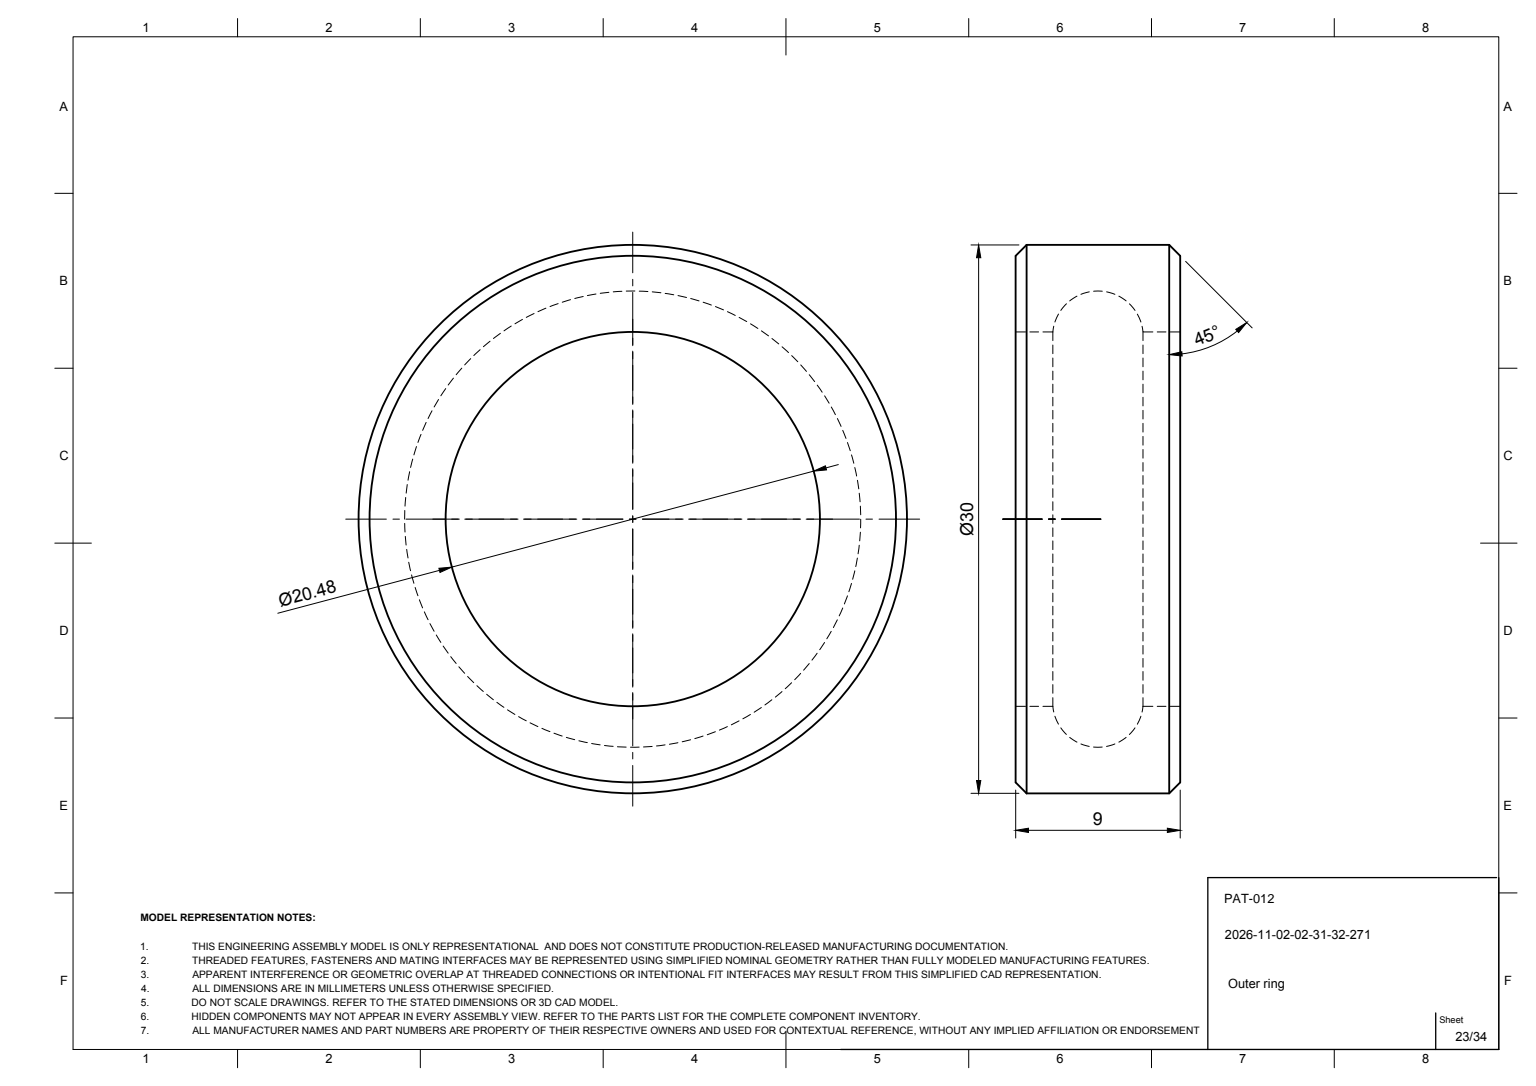
ISO-10303-21;
HEADER;
/* Generated by software containing ST-Developer
 * from STEP Tools, Inc. (www.steptools.com) 
 */

FILE_DESCRIPTION(
/* description */ ('Belt tensioner idler arm'),
/* implementation_level */ '2;1');

FILE_NAME(
/* name */ 'Outer ring.step',
/* time_stamp */ '2026-10-28T03:22:15-07:00',
/* author */ (''),
/* organization */ (''),
/* preprocessor_version */ 'ST-DEVELOPER v20.2',
/* originating_system */ 'Autodesk Translation Framework v15.17.0.0',
/* authorisation */ '');

FILE_SCHEMA (('AUTOMOTIVE_DESIGN { 1 0 10303 214 3 1 1 }'));
ENDSEC;

DATA;
#10=MECHANICAL_DESIGN_GEOMETRIC_PRESENTATION_REPRESENTATION('',(#466),#12779);
#272=TOROIDAL_SURFACE('',#6988,1.,0.247676);
#306=CONICAL_SURFACE('',#6999,1.47,0.785398163397449);
#307=CONICAL_SURFACE('',#7003,1.47,0.785398163397449);
#398=SHAPE_REPRESENTATION_RELATIONSHIP('SRR','None',#12946,#432);
#432=ADVANCED_BREP_SHAPE_REPRESENTATION('',(#506),#12763);
#466=STYLED_ITEM('',(#13184),#506);
#506=MANIFOLD_SOLID_BREP('Body1',#6202);
#629=FACE_BOUND('',#1503,.T.);
#630=FACE_BOUND('',#1508,.T.);
#767=PLANE('',#6996);
#768=PLANE('',#7005);
#1031=FACE_OUTER_BOUND('',#1500,.T.);
#1032=FACE_OUTER_BOUND('',#1501,.T.);
#1033=FACE_OUTER_BOUND('',#1502,.T.);
#1034=FACE_OUTER_BOUND('',#1504,.T.);
#1035=FACE_OUTER_BOUND('',#1505,.T.);
#1036=FACE_OUTER_BOUND('',#1506,.T.);
#1037=FACE_OUTER_BOUND('',#1507,.T.);
#1038=FACE_OUTER_BOUND('',#1509,.T.);
#1500=EDGE_LOOP('',(#4892,#4893,#4894,#4895,#4896,#4897));
#1501=EDGE_LOOP('',(#4898,#4899,#4900,#4901,#4902));
#1502=EDGE_LOOP('',(#4903));
#1503=EDGE_LOOP('',(#4904));
#1504=EDGE_LOOP('',(#4905,#4906,#4907,#4908));
#1505=EDGE_LOOP('',(#4909,#4910,#4911,#4912));
#1506=EDGE_LOOP('',(#4913,#4914,#4915,#4916));
#1507=EDGE_LOOP('',(#4917));
#1508=EDGE_LOOP('',(#4918));
#1509=EDGE_LOOP('',(#4919,#4920,#4921,#4922,#4923));
#1912=LINE('',#11134,#2261);
#1913=LINE('',#11143,#2262);
#1914=LINE('',#11147,#2263);
#1915=LINE('',#11151,#2264);
#1916=LINE('',#11154,#2265);
#2261=VECTOR('',#8426,1.023815);
#2262=VECTOR('',#8437,1.47);
#2263=VECTOR('',#8442,1.5);
#2264=VECTOR('',#8447,1.47);
#2265=VECTOR('',#8452,1.023815);
#2573=CIRCLE('',#6989,1.023815);
#2574=CIRCLE('',#6990,1.023815);
#2575=CIRCLE('',#6991,0.247676);
#2576=CIRCLE('',#6992,1.023815);
#2577=CIRCLE('',#6993,1.023815);
#2578=CIRCLE('',#6995,1.023815);
#2579=CIRCLE('',#6997,1.44);
#2580=CIRCLE('',#6998,1.023815);
#2581=CIRCLE('',#7000,1.5);
#2582=CIRCLE('',#7002,1.5);
#2583=CIRCLE('',#7004,1.44);
#3030=VERTEX_POINT('',#11122);
#3031=VERTEX_POINT('',#11123);
#3032=VERTEX_POINT('',#11126);
#3033=VERTEX_POINT('',#11128);
#3034=VERTEX_POINT('',#11132);
#3035=VERTEX_POINT('',#11136);
#3036=VERTEX_POINT('',#11138);
#3037=VERTEX_POINT('',#11141);
#3038=VERTEX_POINT('',#11145);
#3039=VERTEX_POINT('',#11149);
#3701=EDGE_CURVE('',#3030,#3031,#2573,.T.);
#3702=EDGE_CURVE('',#3031,#3030,#2574,.T.);
#3703=EDGE_CURVE('',#3031,#3032,#2575,.T.);
#3704=EDGE_CURVE('',#3033,#3032,#2576,.T.);
#3705=EDGE_CURVE('',#3032,#3033,#2577,.T.);
#3706=EDGE_CURVE('',#3034,#3034,#2578,.T.);
#3707=EDGE_CURVE('',#3034,#3033,#1912,.T.);
#3708=EDGE_CURVE('',#3035,#3035,#2579,.T.);
#3709=EDGE_CURVE('',#3036,#3036,#2580,.T.);
#3710=EDGE_CURVE('',#3037,#3037,#2581,.T.);
#3711=EDGE_CURVE('',#3037,#3035,#1913,.T.);
#3712=EDGE_CURVE('',#3038,#3038,#2582,.T.);
#3713=EDGE_CURVE('',#3038,#3037,#1914,.T.);
#3714=EDGE_CURVE('',#3039,#3039,#2583,.T.);
#3715=EDGE_CURVE('',#3039,#3038,#1915,.T.);
#3716=EDGE_CURVE('',#3030,#3036,#1916,.T.);
#4892=ORIENTED_EDGE('',*,*,#3701,.F.);
#4893=ORIENTED_EDGE('',*,*,#3702,.F.);
#4894=ORIENTED_EDGE('',*,*,#3703,.T.);
#4895=ORIENTED_EDGE('',*,*,#3704,.F.);
#4896=ORIENTED_EDGE('',*,*,#3705,.F.);
#4897=ORIENTED_EDGE('',*,*,#3703,.F.);
#4898=ORIENTED_EDGE('',*,*,#3706,.T.);
#4899=ORIENTED_EDGE('',*,*,#3707,.T.);
#4900=ORIENTED_EDGE('',*,*,#3704,.T.);
#4901=ORIENTED_EDGE('',*,*,#3705,.T.);
#4902=ORIENTED_EDGE('',*,*,#3707,.F.);
#4903=ORIENTED_EDGE('',*,*,#3708,.F.);
#4904=ORIENTED_EDGE('',*,*,#3709,.T.);
#4905=ORIENTED_EDGE('',*,*,#3710,.F.);
#4906=ORIENTED_EDGE('',*,*,#3711,.T.);
#4907=ORIENTED_EDGE('',*,*,#3708,.T.);
#4908=ORIENTED_EDGE('',*,*,#3711,.F.);
#4909=ORIENTED_EDGE('',*,*,#3712,.F.);
#4910=ORIENTED_EDGE('',*,*,#3713,.T.);
#4911=ORIENTED_EDGE('',*,*,#3710,.T.);
#4912=ORIENTED_EDGE('',*,*,#3713,.F.);
#4913=ORIENTED_EDGE('',*,*,#3714,.F.);
#4914=ORIENTED_EDGE('',*,*,#3715,.T.);
#4915=ORIENTED_EDGE('',*,*,#3712,.T.);
#4916=ORIENTED_EDGE('',*,*,#3715,.F.);
#4917=ORIENTED_EDGE('',*,*,#3714,.T.);
#4918=ORIENTED_EDGE('',*,*,#3706,.F.);
#4919=ORIENTED_EDGE('',*,*,#3701,.T.);
#4920=ORIENTED_EDGE('',*,*,#3702,.T.);
#4921=ORIENTED_EDGE('',*,*,#3716,.T.);
#4922=ORIENTED_EDGE('',*,*,#3709,.F.);
#4923=ORIENTED_EDGE('',*,*,#3716,.F.);
#5737=CYLINDRICAL_SURFACE('',#6994,1.023815);
#5738=CYLINDRICAL_SURFACE('',#7001,1.5);
#5739=CYLINDRICAL_SURFACE('',#7006,1.023815);
#6008=ADVANCED_FACE('',(#1031),#272,.F.);
#6009=ADVANCED_FACE('',(#1032),#5737,.F.);
#6010=ADVANCED_FACE('',(#1033,#629),#767,.T.);
#6011=ADVANCED_FACE('',(#1034),#306,.T.);
#6012=ADVANCED_FACE('',(#1035),#5738,.T.);
#6013=ADVANCED_FACE('',(#1036),#307,.T.);
#6014=ADVANCED_FACE('',(#1037,#630),#768,.T.);
#6015=ADVANCED_FACE('',(#1038),#5739,.F.);
#6202=CLOSED_SHELL('',(#6008,#6009,#6010,#6011,#6012,#6013,#6014,#6015));
#6987=AXIS2_PLACEMENT_3D('',#11120,#8408,#8409);
#6988=AXIS2_PLACEMENT_3D('',#11121,#8410,#8411);
#6989=AXIS2_PLACEMENT_3D('',#11124,#8412,#8413);
#6990=AXIS2_PLACEMENT_3D('',#11125,#8414,#8415);
#6991=AXIS2_PLACEMENT_3D('',#11127,#8416,#8417);
#6992=AXIS2_PLACEMENT_3D('',#11129,#8418,#8419);
#6993=AXIS2_PLACEMENT_3D('',#11130,#8420,#8421);
#6994=AXIS2_PLACEMENT_3D('',#11131,#8422,#8423);
#6995=AXIS2_PLACEMENT_3D('',#11133,#8424,#8425);
#6996=AXIS2_PLACEMENT_3D('',#11135,#8427,#8428);
#6997=AXIS2_PLACEMENT_3D('',#11137,#8429,#8430);
#6998=AXIS2_PLACEMENT_3D('',#11139,#8431,#8432);
#6999=AXIS2_PLACEMENT_3D('',#11140,#8433,#8434);
#7000=AXIS2_PLACEMENT_3D('',#11142,#8435,#8436);
#7001=AXIS2_PLACEMENT_3D('',#11144,#8438,#8439);
#7002=AXIS2_PLACEMENT_3D('',#11146,#8440,#8441);
#7003=AXIS2_PLACEMENT_3D('',#11148,#8443,#8444);
#7004=AXIS2_PLACEMENT_3D('',#11150,#8445,#8446);
#7005=AXIS2_PLACEMENT_3D('',#11152,#8448,#8449);
#7006=AXIS2_PLACEMENT_3D('',#11153,#8450,#8451);
#8408=DIRECTION('axis',(0.,0.,1.));
#8409=DIRECTION('refdir',(1.,0.,0.));
#8410=DIRECTION('center_axis',(0.,-1.,0.));
#8411=DIRECTION('ref_axis',(0.,0.,-1.));
#8412=DIRECTION('center_axis',(0.,-1.,0.));
#8413=DIRECTION('ref_axis',(1.,0.,0.));
#8414=DIRECTION('center_axis',(0.,-1.,0.));
#8415=DIRECTION('ref_axis',(1.,0.,0.));
#8416=DIRECTION('center_axis',(1.,0.,1.22464679914735E-16));
#8417=DIRECTION('ref_axis',(-1.22464679914735E-16,0.,1.));
#8418=DIRECTION('center_axis',(0.,1.,0.));
#8419=DIRECTION('ref_axis',(1.,0.,0.));
#8420=DIRECTION('center_axis',(0.,1.,0.));
#8421=DIRECTION('ref_axis',(1.,0.,0.));
#8422=DIRECTION('center_axis',(0.,-1.,0.));
#8423=DIRECTION('ref_axis',(1.,0.,0.));
#8424=DIRECTION('center_axis',(0.,-1.,0.));
#8425=DIRECTION('ref_axis',(1.,0.,0.));
#8426=DIRECTION('',(0.,1.,0.));
#8427=DIRECTION('center_axis',(0.,1.,0.));
#8428=DIRECTION('ref_axis',(0.,0.,1.));
#8429=DIRECTION('center_axis',(0.,-1.,0.));
#8430=DIRECTION('ref_axis',(1.,0.,0.));
#8431=DIRECTION('center_axis',(0.,-1.,0.));
#8432=DIRECTION('ref_axis',(1.,0.,0.));
#8433=DIRECTION('center_axis',(0.,-1.,0.));
#8434=DIRECTION('ref_axis',(1.,0.,0.));
#8435=DIRECTION('center_axis',(0.,-1.,0.));
#8436=DIRECTION('ref_axis',(1.,0.,0.));
#8437=DIRECTION('',(0.707106781186548,0.707106781186547,8.65956056235494E-17));
#8438=DIRECTION('center_axis',(0.,-1.,0.));
#8439=DIRECTION('ref_axis',(1.,0.,0.));
#8440=DIRECTION('center_axis',(0.,-1.,0.));
#8441=DIRECTION('ref_axis',(1.,0.,0.));
#8442=DIRECTION('',(0.,1.,0.));
#8443=DIRECTION('center_axis',(0.,1.,0.));
#8444=DIRECTION('ref_axis',(1.,0.,0.));
#8445=DIRECTION('center_axis',(0.,-1.,0.));
#8446=DIRECTION('ref_axis',(1.,0.,0.));
#8447=DIRECTION('',(-0.707106781186548,0.707106781186547,-8.65956056235494E-17));
#8448=DIRECTION('center_axis',(0.,-1.,0.));
#8449=DIRECTION('ref_axis',(0.,0.,-1.));
#8450=DIRECTION('center_axis',(0.,-1.,0.));
#8451=DIRECTION('ref_axis',(1.,0.,0.));
#8452=DIRECTION('',(0.,1.,0.));
#11120=CARTESIAN_POINT('',(0.,0.,0.));
#11121=CARTESIAN_POINT('Origin',(0.,0.,0.));
#11122=CARTESIAN_POINT('',(-1.023815,0.246528389340863,-1.25381176266905E-16));
#11123=CARTESIAN_POINT('',(-1.25381176266905E-16,0.246528389340863,1.023815));
#11124=CARTESIAN_POINT('Origin',(0.,0.246528389340863,0.));
#11125=CARTESIAN_POINT('Origin',(0.,0.246528389340863,0.));
#11126=CARTESIAN_POINT('',(-1.25381176266905E-16,-0.246528389340863,1.023815));
#11127=CARTESIAN_POINT('Origin',(-1.22464679914735E-16,0.,1.));
#11128=CARTESIAN_POINT('',(-1.023815,-0.246528389340863,1.25381176266905E-16));
#11129=CARTESIAN_POINT('Origin',(0.,-0.246528389340863,0.));
#11130=CARTESIAN_POINT('Origin',(0.,-0.246528389340863,0.));
#11131=CARTESIAN_POINT('Origin',(0.,0.,0.));
#11132=CARTESIAN_POINT('',(-1.023815,-0.45,-1.25381176266905E-16));
#11133=CARTESIAN_POINT('Origin',(0.,-0.45,0.));
#11134=CARTESIAN_POINT('',(-1.023815,0.,-1.25381176266905E-16));
#11135=CARTESIAN_POINT('Origin',(1.44,0.45,0.));
#11136=CARTESIAN_POINT('',(-1.44,0.45,-1.76349139077219E-16));
#11137=CARTESIAN_POINT('Origin',(0.,0.45,0.));
#11138=CARTESIAN_POINT('',(-1.023815,0.45,-1.25381176266905E-16));
#11139=CARTESIAN_POINT('Origin',(0.,0.45,0.));
#11140=CARTESIAN_POINT('Origin',(0.,0.42,0.));
#11141=CARTESIAN_POINT('',(-1.5,0.39,-1.83697019872103E-16));
#11142=CARTESIAN_POINT('Origin',(0.,0.39,0.));
#11143=CARTESIAN_POINT('',(-1.47,0.42,-1.80023079474661E-16));
#11144=CARTESIAN_POINT('Origin',(0.,0.,0.));
#11145=CARTESIAN_POINT('',(-1.5,-0.39,-1.83697019872103E-16));
#11146=CARTESIAN_POINT('Origin',(0.,-0.39,0.));
#11147=CARTESIAN_POINT('',(-1.5,0.,-1.83697019872103E-16));
#11148=CARTESIAN_POINT('Origin',(0.,-0.42,0.));
#11149=CARTESIAN_POINT('',(-1.44,-0.45,-1.76349139077219E-16));
#11150=CARTESIAN_POINT('Origin',(0.,-0.45,0.));
#11151=CARTESIAN_POINT('',(-1.47,-0.42,-1.80023079474661E-16));
#11152=CARTESIAN_POINT('Origin',(1.023815,-0.45,0.));
#11153=CARTESIAN_POINT('Origin',(0.,0.,0.));
#11154=CARTESIAN_POINT('',(-1.023815,0.,-1.25381176266905E-16));
#12723=UNCERTAINTY_MEASURE_WITH_UNIT(LENGTH_MEASURE(0.001),#12780,
'DISTANCE_ACCURACY_VALUE',
'Maximum model space distance between geometric entities at asserted c
onnectivities');
#12739=UNCERTAINTY_MEASURE_WITH_UNIT(LENGTH_MEASURE(0.001),#12780,
'DISTANCE_ACCURACY_VALUE',
'Maximum model space distance between geometric entities at asserted c
onnectivities');
#12763=(
GEOMETRIC_REPRESENTATION_CONTEXT(3)
GLOBAL_UNCERTAINTY_ASSIGNED_CONTEXT((#12723))
GLOBAL_UNIT_ASSIGNED_CONTEXT((#12780,#12782,#12783))
REPRESENTATION_CONTEXT('','3D')
);
#12779=(
GEOMETRIC_REPRESENTATION_CONTEXT(3)
GLOBAL_UNCERTAINTY_ASSIGNED_CONTEXT((#12739))
GLOBAL_UNIT_ASSIGNED_CONTEXT((#12780,#12782,#12783))
REPRESENTATION_CONTEXT('','3D')
);
#12780=(
LENGTH_UNIT()
NAMED_UNIT(*)
SI_UNIT(.CENTI.,.METRE.)
);
#12782=(
NAMED_UNIT(*)
PLANE_ANGLE_UNIT()
SI_UNIT($,.RADIAN.)
);
#12783=(
NAMED_UNIT(*)
SI_UNIT($,.STERADIAN.)
SOLID_ANGLE_UNIT()
);
#12807=SHAPE_DEFINITION_REPRESENTATION(#12846,#12946);
#12846=PRODUCT_DEFINITION_SHAPE('',$,#12986);
#12946=SHAPE_REPRESENTATION('',(#6987),#12763);
#12962=PRODUCT_DEFINITION_CONTEXT('part definition',#13081,'design');
#12986=PRODUCT_DEFINITION('Outer ring','Outer ring',#13025,#12962);
#13025=PRODUCT_DEFINITION_FORMATION('',$,#13106);
#13081=APPLICATION_CONTEXT(
'Core Data for Automotive Mechanical Design Process');
#13082=PRODUCT_CONTEXT('part definition',#13081,'mechanical');
#13106=PRODUCT('Outer ring','Outer ring','Outer ring',(#13082));
#13178=COLOUR_RGB('Grey',0.48,0.52,0.57);
#13179=FILL_AREA_STYLE_COLOUR('',#13178);
#13180=FILL_AREA_STYLE('',(#13179));
#13181=SURFACE_STYLE_FILL_AREA(#13180);
#13182=SURFACE_SIDE_STYLE('',(#13181));
#13183=SURFACE_STYLE_USAGE(.BOTH.,#13182);
#13184=PRESENTATION_STYLE_ASSIGNMENT((#13183));
ENDSEC;
END-ISO-10303-21;
